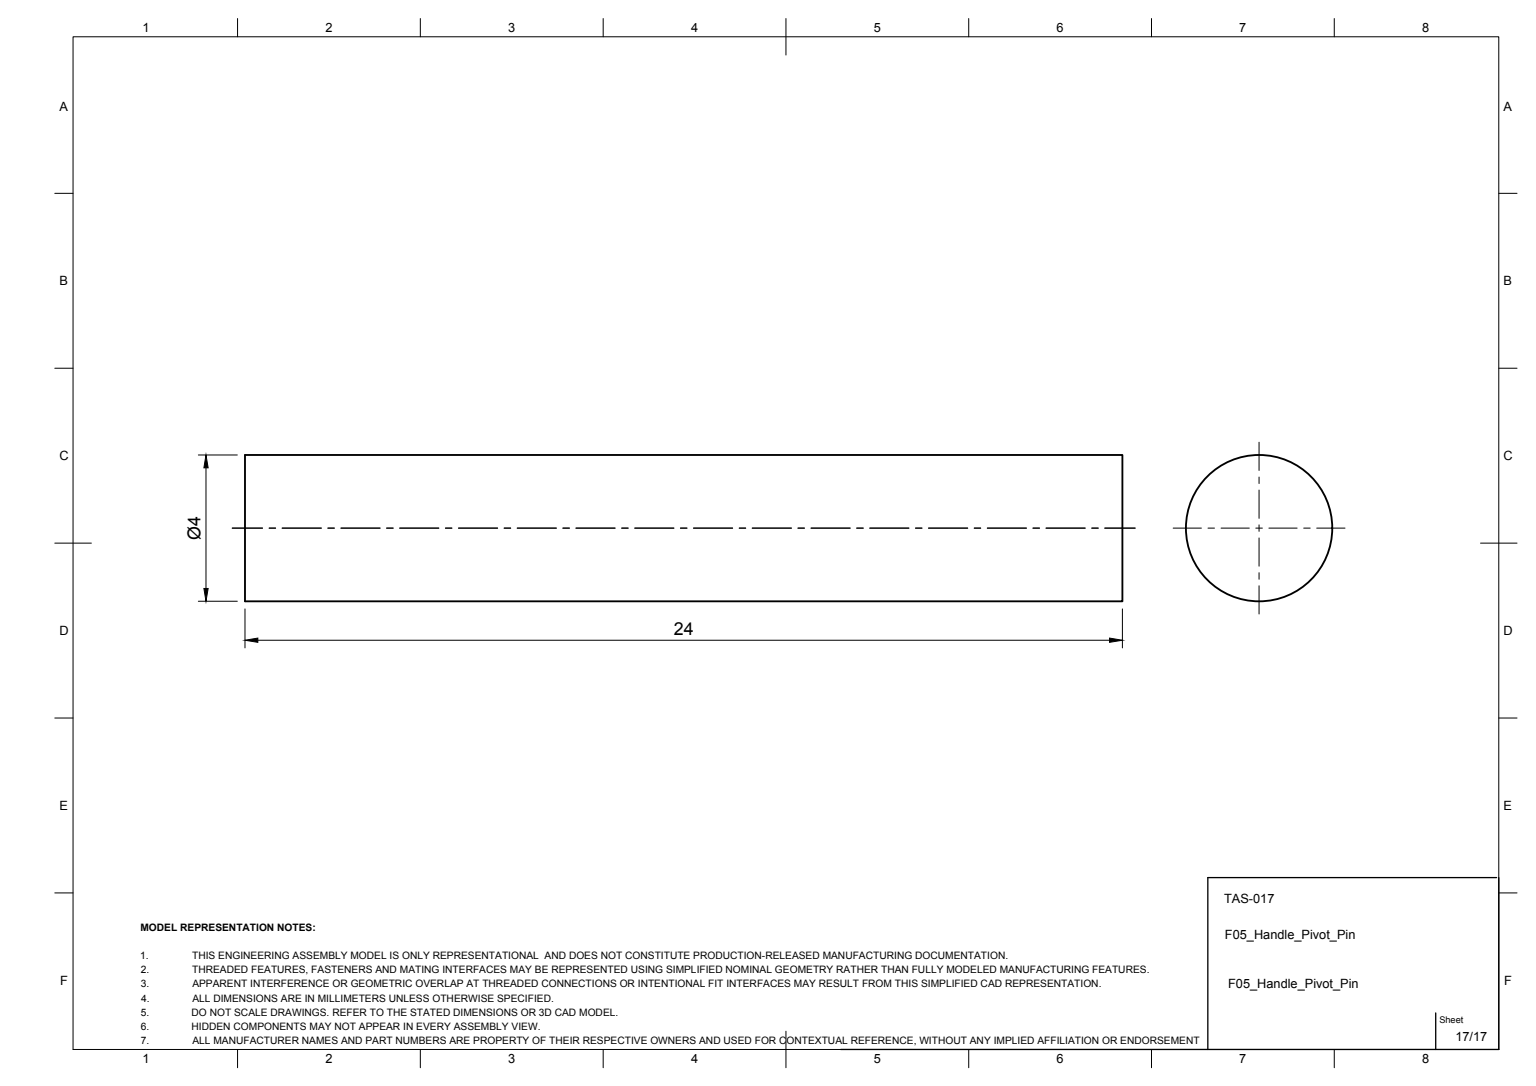
ISO-10303-21;
HEADER;
/* Generated by software containing ST-Developer
 * from STEP Tools, Inc. (www.steptools.com) 
 */

FILE_DESCRIPTION(
/* description */ ('STEP AP203'),
/* implementation_level */ '2;1');

FILE_NAME(
/* name */ 'F05_Handle_Pivot_Pin.step',
/* time_stamp */ '2026-11-15T15:04:01-08:00',
/* author */ (''),
/* organization */ (''),
/* preprocessor_version */ 'ST-DEVELOPER v20.2',
/* originating_system */ 'Autodesk Translation Framework v15.17.0.0',
/* authorisation */ '');

FILE_SCHEMA (('AUTOMOTIVE_DESIGN { 1 0 10303 214 3 1 1 }'));
ENDSEC;

DATA;
#10=MECHANICAL_DESIGN_GEOMETRIC_PRESENTATION_REPRESENTATION('',(#295),#16598);
#217=SHAPE_REPRESENTATION_RELATIONSHIP('SRR','None',#16711,#241);
#241=ADVANCED_BREP_SHAPE_REPRESENTATION('',(#265),#16587);
#265=MANIFOLD_SOLID_BREP('Body1',#9800);
#295=STYLED_ITEM('',(#16830),#265);
#631=PLANE('',#10444);
#632=PLANE('',#10445);
#1158=FACE_OUTER_BOUND('',#1765,.T.);
#1159=FACE_OUTER_BOUND('',#1766,.T.);
#1160=FACE_OUTER_BOUND('',#1767,.T.);
#1765=EDGE_LOOP('',(#7761,#7762,#7763,#7764));
#1766=EDGE_LOOP('',(#7765));
#1767=EDGE_LOOP('',(#7766));
#2609=LINE('',#15020,#3657);
#3657=VECTOR('',#12135,2.);
#4326=CIRCLE('',#10442,2.);
#4327=CIRCLE('',#10443,2.);
#4842=VERTEX_POINT('',#15017);
#4843=VERTEX_POINT('',#15019);
#5893=EDGE_CURVE('',#4842,#4842,#4326,.T.);
#5894=EDGE_CURVE('',#4842,#4843,#2609,.T.);
#5895=EDGE_CURVE('',#4843,#4843,#4327,.T.);
#7761=ORIENTED_EDGE('',*,*,#5893,.T.);
#7762=ORIENTED_EDGE('',*,*,#5894,.T.);
#7763=ORIENTED_EDGE('',*,*,#5895,.F.);
#7764=ORIENTED_EDGE('',*,*,#5894,.F.);
#7765=ORIENTED_EDGE('',*,*,#5895,.T.);
#7766=ORIENTED_EDGE('',*,*,#5893,.F.);
#9214=CYLINDRICAL_SURFACE('',#10441,2.);
#9483=ADVANCED_FACE('',(#1158),#9214,.T.);
#9484=ADVANCED_FACE('',(#1159),#631,.T.);
#9485=ADVANCED_FACE('',(#1160),#632,.F.);
#9800=CLOSED_SHELL('',(#9483,#9484,#9485));
#10440=AXIS2_PLACEMENT_3D('',#15015,#12129,#12130);
#10441=AXIS2_PLACEMENT_3D('',#15016,#12131,#12132);
#10442=AXIS2_PLACEMENT_3D('',#15018,#12133,#12134);
#10443=AXIS2_PLACEMENT_3D('',#15021,#12136,#12137);
#10444=AXIS2_PLACEMENT_3D('',#15022,#12138,#12139);
#10445=AXIS2_PLACEMENT_3D('',#15023,#12140,#12141);
#12129=DIRECTION('axis',(0.,0.,1.));
#12130=DIRECTION('refdir',(1.,0.,0.));
#12131=DIRECTION('center_axis',(0.,0.,-1.));
#12132=DIRECTION('ref_axis',(-1.,0.,0.));
#12133=DIRECTION('center_axis',(0.,0.,1.));
#12134=DIRECTION('ref_axis',(1.,0.,0.));
#12135=DIRECTION('',(0.,0.,1.));
#12136=DIRECTION('center_axis',(0.,0.,1.));
#12137=DIRECTION('ref_axis',(1.,0.,0.));
#12138=DIRECTION('center_axis',(0.,0.,1.));
#12139=DIRECTION('ref_axis',(1.,0.,0.));
#12140=DIRECTION('center_axis',(0.,0.,1.));
#12141=DIRECTION('ref_axis',(1.,0.,0.));
#15015=CARTESIAN_POINT('',(0.,0.,0.));
#15016=CARTESIAN_POINT('Origin',(0.,0.,12.));
#15017=CARTESIAN_POINT('',(2.,-2.44929359829471E-16,-12.));
#15018=CARTESIAN_POINT('Origin',(0.,0.,-12.));
#15019=CARTESIAN_POINT('',(2.,-2.44929359829471E-16,12.));
#15020=CARTESIAN_POINT('',(2.,-2.44929359829471E-16,12.));
#15021=CARTESIAN_POINT('Origin',(0.,0.,12.));
#15022=CARTESIAN_POINT('Origin',(0.,0.,12.));
#15023=CARTESIAN_POINT('Origin',(0.,0.,-12.));
#16561=UNCERTAINTY_MEASURE_WITH_UNIT(LENGTH_MEASURE(0.01),#16599,
'DISTANCE_ACCURACY_VALUE',
'Maximum model space distance between geometric entities at asserted c
onnectivities');
#16572=UNCERTAINTY_MEASURE_WITH_UNIT(LENGTH_MEASURE(0.01),#16599,
'DISTANCE_ACCURACY_VALUE',
'Maximum model space distance between geometric entities at asserted c
onnectivities');
#16587=(
GEOMETRIC_REPRESENTATION_CONTEXT(3)
GLOBAL_UNCERTAINTY_ASSIGNED_CONTEXT((#16561))
GLOBAL_UNIT_ASSIGNED_CONTEXT((#16599,#16601,#16602))
REPRESENTATION_CONTEXT('','3D')
);
#16598=(
GEOMETRIC_REPRESENTATION_CONTEXT(3)
GLOBAL_UNCERTAINTY_ASSIGNED_CONTEXT((#16572))
GLOBAL_UNIT_ASSIGNED_CONTEXT((#16599,#16601,#16602))
REPRESENTATION_CONTEXT('','3D')
);
#16599=(
LENGTH_UNIT()
NAMED_UNIT(*)
SI_UNIT(.MILLI.,.METRE.)
);
#16601=(
NAMED_UNIT(*)
PLANE_ANGLE_UNIT()
SI_UNIT($,.RADIAN.)
);
#16602=(
NAMED_UNIT(*)
SI_UNIT($,.STERADIAN.)
SOLID_ANGLE_UNIT()
);
#16617=SHAPE_DEFINITION_REPRESENTATION(#16642,#16711);
#16642=PRODUCT_DEFINITION_SHAPE('',$,#16737);
#16711=SHAPE_REPRESENTATION('',(#10440),#16587);
#16722=PRODUCT_DEFINITION_CONTEXT('part definition',#16799,'design');
#16737=PRODUCT_DEFINITION('F05_Handle_Pivot_Pin','F05_Handle_Pivot_Pin',
#16762,#16722);
#16762=PRODUCT_DEFINITION_FORMATION('',$,#16815);
#16799=APPLICATION_CONTEXT(
'Core Data for Automotive Mechanical Design Process');
#16800=PRODUCT_CONTEXT('part definition',#16799,'mechanical');
#16815=PRODUCT('F05_Handle_Pivot_Pin','F05_Handle_Pivot_Pin',$,(#16800));
#16830=PRESENTATION_STYLE_ASSIGNMENT((#16839));
#16839=SURFACE_STYLE_USAGE(.BOTH.,#16848);
#16848=SURFACE_SIDE_STYLE('',(#16857));
#16857=SURFACE_STYLE_FILL_AREA(#16866);
#16866=FILL_AREA_STYLE('Dark Blue',(#16875));
#16875=FILL_AREA_STYLE_COLOUR('Dark Blue',#16884);
#16884=COLOUR_RGB('Dark Blue',0.,0.125490196078431,0.376470588235294);
ENDSEC;
END-ISO-10303-21;
